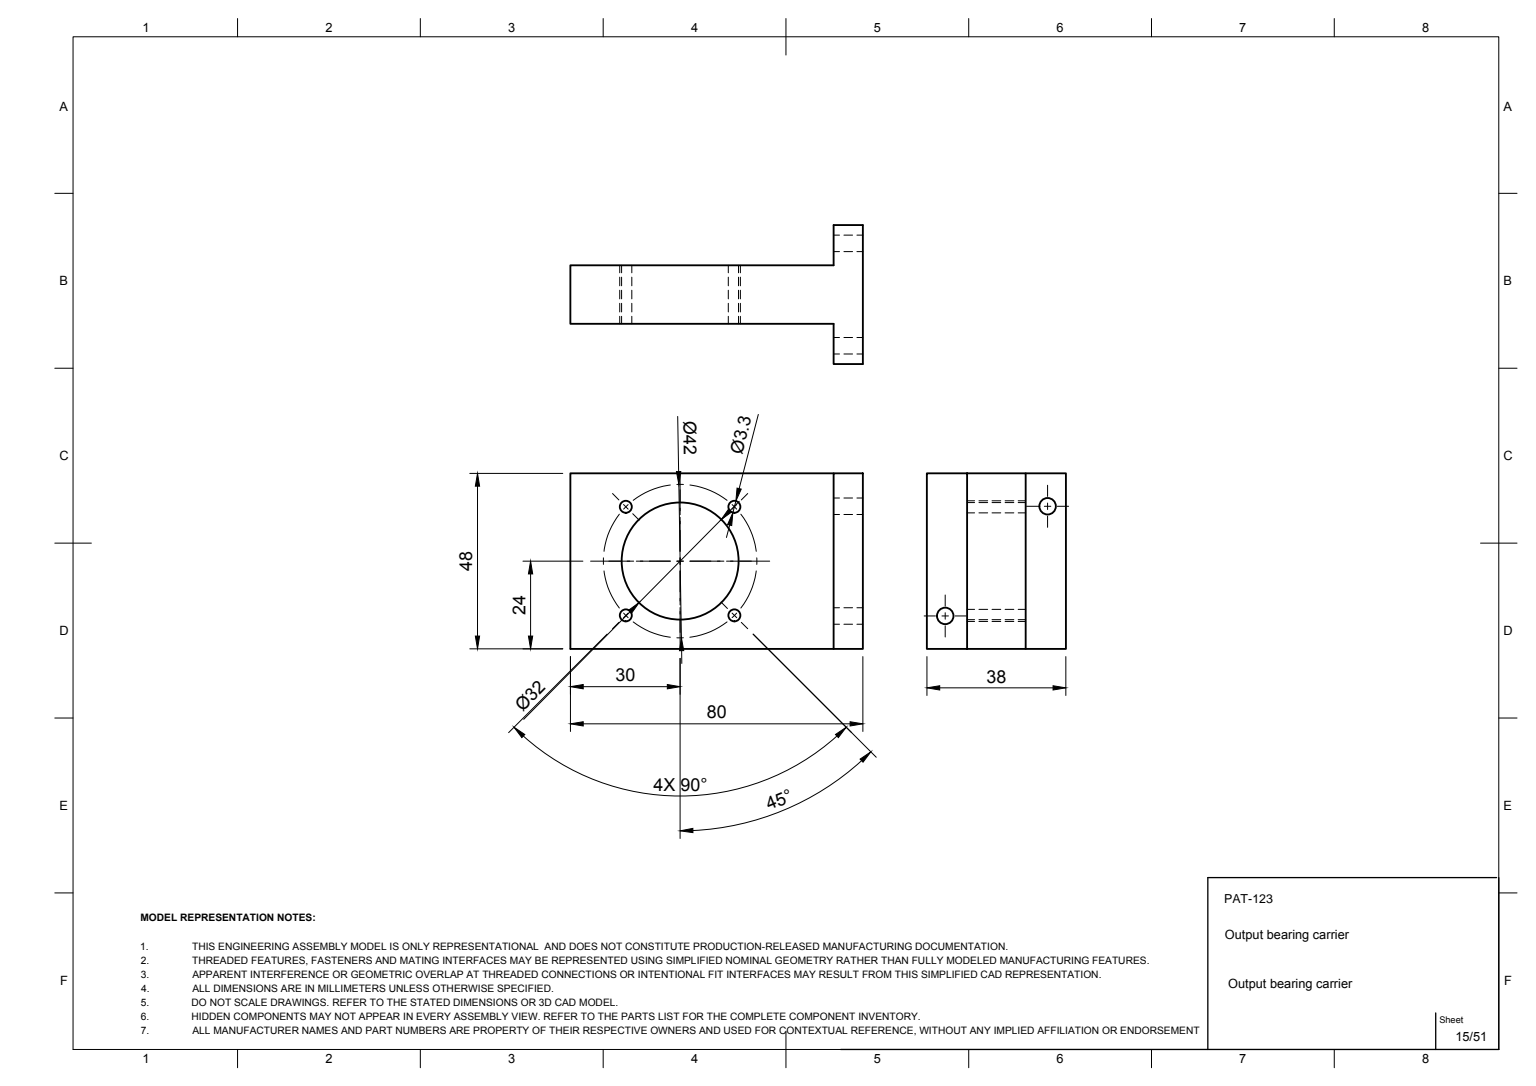
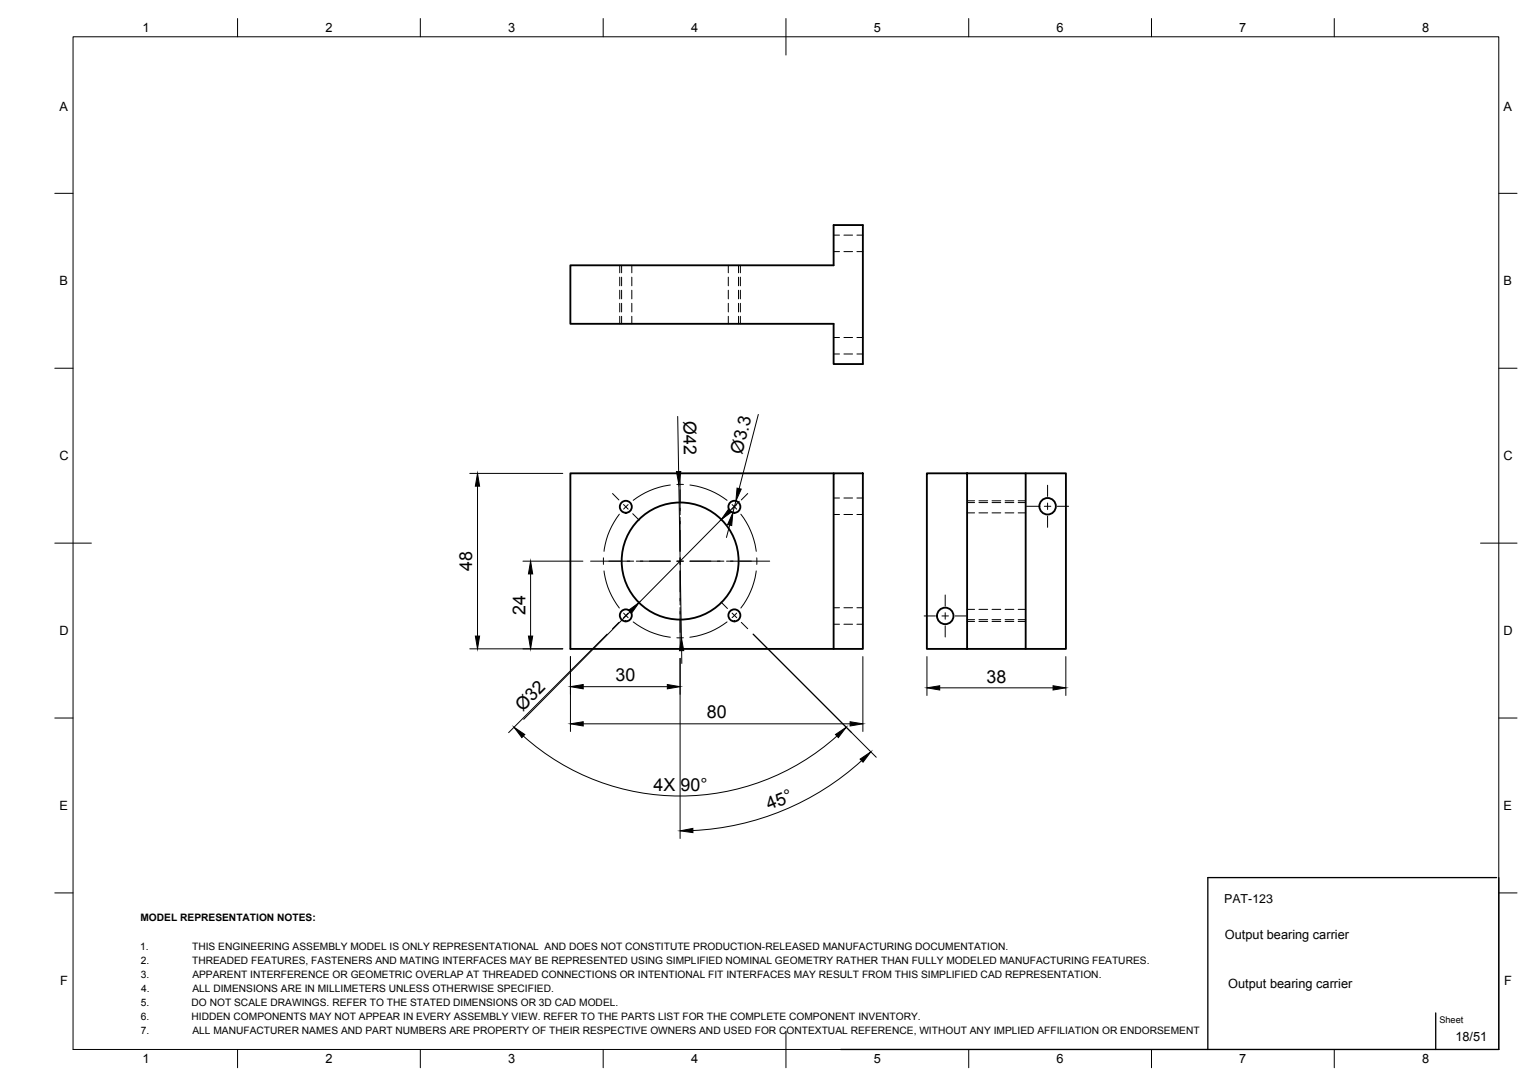
ISO-10303-21;
HEADER;
/* Generated by software containing ST-Developer
 * from STEP Tools, Inc. (www.steptools.com) 
 */

FILE_DESCRIPTION(
/* description */ ('Worm-less right-angle friction wheel drive'),
/* implementation_level */ '2;1');

FILE_NAME(
/* name */ 'Output bearing carrier.step',
/* time_stamp */ '2026-10-28T03:22:36-07:00',
/* author */ (''),
/* organization */ (''),
/* preprocessor_version */ 'ST-DEVELOPER v20.2',
/* originating_system */ 'Autodesk Translation Framework v15.17.0.0',
/* authorisation */ '');

FILE_SCHEMA (('AUTOMOTIVE_DESIGN { 1 0 10303 214 3 1 1 }'));
ENDSEC;

DATA;
#10=MECHANICAL_DESIGN_GEOMETRIC_PRESENTATION_REPRESENTATION('',(#621),#17046);
#527=SHAPE_REPRESENTATION_RELATIONSHIP('SRR','None',#17270,#574);
#574=ADVANCED_BREP_SHAPE_REPRESENTATION('',(#675),#17006);
#621=STYLED_ITEM('',(#17591),#675);
#675=MANIFOLD_SOLID_BREP('Body1',#8176);
#823=FACE_BOUND('',#1918,.T.);
#824=FACE_BOUND('',#1920,.T.);
#825=FACE_BOUND('',#1925,.T.);
#826=FACE_BOUND('',#1926,.T.);
#827=FACE_BOUND('',#1927,.T.);
#828=FACE_BOUND('',#1928,.T.);
#829=FACE_BOUND('',#1929,.T.);
#830=FACE_BOUND('',#1932,.T.);
#831=FACE_BOUND('',#1933,.T.);
#832=FACE_BOUND('',#1934,.T.);
#833=FACE_BOUND('',#1935,.T.);
#834=FACE_BOUND('',#1936,.T.);
#835=FACE_BOUND('',#1939,.T.);
#836=FACE_BOUND('',#1940,.T.);
#1016=PLANE('',#9032);
#1017=PLANE('',#9033);
#1018=PLANE('',#9034);
#1019=PLANE('',#9035);
#1020=PLANE('',#9036);
#1021=PLANE('',#9037);
#1022=PLANE('',#9038);
#1023=PLANE('',#9039);
#1024=PLANE('',#9040);
#1025=PLANE('',#9041);
#1336=FACE_OUTER_BOUND('',#1910,.T.);
#1337=FACE_OUTER_BOUND('',#1911,.T.);
#1338=FACE_OUTER_BOUND('',#1912,.T.);
#1339=FACE_OUTER_BOUND('',#1913,.T.);
#1340=FACE_OUTER_BOUND('',#1914,.T.);
#1341=FACE_OUTER_BOUND('',#1915,.T.);
#1342=FACE_OUTER_BOUND('',#1916,.T.);
#1343=FACE_OUTER_BOUND('',#1917,.T.);
#1344=FACE_OUTER_BOUND('',#1919,.T.);
#1345=FACE_OUTER_BOUND('',#1921,.T.);
#1346=FACE_OUTER_BOUND('',#1922,.T.);
#1347=FACE_OUTER_BOUND('',#1923,.T.);
#1348=FACE_OUTER_BOUND('',#1924,.T.);
#1349=FACE_OUTER_BOUND('',#1930,.T.);
#1350=FACE_OUTER_BOUND('',#1931,.T.);
#1351=FACE_OUTER_BOUND('',#1937,.T.);
#1352=FACE_OUTER_BOUND('',#1938,.T.);
#1910=EDGE_LOOP('',(#6158,#6159,#6160,#6161));
#1911=EDGE_LOOP('',(#6162,#6163,#6164,#6165));
#1912=EDGE_LOOP('',(#6166,#6167,#6168,#6169));
#1913=EDGE_LOOP('',(#6170,#6171,#6172,#6173));
#1914=EDGE_LOOP('',(#6174,#6175,#6176,#6177));
#1915=EDGE_LOOP('',(#6178,#6179,#6180,#6181));
#1916=EDGE_LOOP('',(#6182,#6183,#6184,#6185));
#1917=EDGE_LOOP('',(#6186,#6187,#6188,#6189));
#1918=EDGE_LOOP('',(#6190));
#1919=EDGE_LOOP('',(#6191,#6192,#6193,#6194));
#1920=EDGE_LOOP('',(#6195));
#1921=EDGE_LOOP('',(#6196,#6197,#6198,#6199));
#1922=EDGE_LOOP('',(#6200,#6201,#6202,#6203));
#1923=EDGE_LOOP('',(#6204,#6205,#6206,#6207,#6208,#6209,#6210,#6211));
#1924=EDGE_LOOP('',(#6212,#6213,#6214,#6215));
#1925=EDGE_LOOP('',(#6216));
#1926=EDGE_LOOP('',(#6217));
#1927=EDGE_LOOP('',(#6218));
#1928=EDGE_LOOP('',(#6219));
#1929=EDGE_LOOP('',(#6220));
#1930=EDGE_LOOP('',(#6221,#6222,#6223,#6224,#6225,#6226,#6227,#6228));
#1931=EDGE_LOOP('',(#6229,#6230,#6231,#6232));
#1932=EDGE_LOOP('',(#6233));
#1933=EDGE_LOOP('',(#6234));
#1934=EDGE_LOOP('',(#6235));
#1935=EDGE_LOOP('',(#6236));
#1936=EDGE_LOOP('',(#6237));
#1937=EDGE_LOOP('',(#6238,#6239,#6240,#6241));
#1938=EDGE_LOOP('',(#6242,#6243,#6244,#6245));
#1939=EDGE_LOOP('',(#6246));
#1940=EDGE_LOOP('',(#6247));
#2561=LINE('',#13040,#3101);
#2562=LINE('',#13046,#3102);
#2563=LINE('',#13052,#3103);
#2564=LINE('',#13058,#3104);
#2565=LINE('',#13064,#3105);
#2566=LINE('',#13070,#3106);
#2567=LINE('',#13076,#3107);
#2568=LINE('',#13081,#3108);
#2569=LINE('',#13083,#3109);
#2570=LINE('',#13085,#3110);
#2571=LINE('',#13086,#3111);
#2572=LINE('',#13090,#3112);
#2573=LINE('',#13092,#3113);
#2574=LINE('',#13094,#3114);
#2575=LINE('',#13095,#3115);
#2576=LINE('',#13098,#3116);
#2577=LINE('',#13100,#3117);
#2578=LINE('',#13101,#3118);
#2579=LINE('',#13104,#3119);
#2580=LINE('',#13106,#3120);
#2581=LINE('',#13107,#3121);
#2582=LINE('',#13110,#3122);
#2583=LINE('',#13112,#3123);
#2584=LINE('',#13113,#3124);
#2585=LINE('',#13114,#3125);
#2586=LINE('',#13117,#3126);
#2587=LINE('',#13118,#3127);
#2588=LINE('',#13121,#3128);
#2589=LINE('',#13122,#3129);
#2590=LINE('',#13123,#3130);
#2591=LINE('',#13125,#3131);
#3101=VECTOR('',#10499,0.165);
#3102=VECTOR('',#10506,0.164999999999999);
#3103=VECTOR('',#10513,0.164999999999999);
#3104=VECTOR('',#10520,0.165);
#3105=VECTOR('',#10527,1.6);
#3106=VECTOR('',#10534,0.225);
#3107=VECTOR('',#10541,0.225);
#3108=VECTOR('',#10546,1.);
#3109=VECTOR('',#10547,1.);
#3110=VECTOR('',#10548,1.);
#3111=VECTOR('',#10549,1.);
#3112=VECTOR('',#10552,1.);
#3113=VECTOR('',#10553,1.);
#3114=VECTOR('',#10554,1.);
#3115=VECTOR('',#10555,1.);
#3116=VECTOR('',#10558,1.);
#3117=VECTOR('',#10559,1.);
#3118=VECTOR('',#10560,1.);
#3119=VECTOR('',#10563,1.);
#3120=VECTOR('',#10564,1.);
#3121=VECTOR('',#10565,1.);
#3122=VECTOR('',#10568,1.);
#3123=VECTOR('',#10569,1.);
#3124=VECTOR('',#10570,1.);
#3125=VECTOR('',#10571,1.);
#3126=VECTOR('',#10574,1.);
#3127=VECTOR('',#10575,1.);
#3128=VECTOR('',#10578,1.);
#3129=VECTOR('',#10579,1.);
#3130=VECTOR('',#10580,1.);
#3131=VECTOR('',#10583,1.);
#3585=CIRCLE('',#9012,0.165);
#3586=CIRCLE('',#9013,0.165);
#3587=CIRCLE('',#9015,0.164999999999999);
#3588=CIRCLE('',#9016,0.164999999999999);
#3589=CIRCLE('',#9018,0.164999999999999);
#3590=CIRCLE('',#9019,0.164999999999999);
#3591=CIRCLE('',#9021,0.165);
#3592=CIRCLE('',#9022,0.165);
#3593=CIRCLE('',#9024,1.6);
#3594=CIRCLE('',#9025,1.6);
#3595=CIRCLE('',#9027,0.225);
#3596=CIRCLE('',#9028,0.225);
#3597=CIRCLE('',#9030,0.225);
#3598=CIRCLE('',#9031,0.225);
#4077=VERTEX_POINT('',#13037);
#4078=VERTEX_POINT('',#13039);
#4079=VERTEX_POINT('',#13043);
#4080=VERTEX_POINT('',#13045);
#4081=VERTEX_POINT('',#13049);
#4082=VERTEX_POINT('',#13051);
#4083=VERTEX_POINT('',#13055);
#4084=VERTEX_POINT('',#13057);
#4085=VERTEX_POINT('',#13061);
#4086=VERTEX_POINT('',#13063);
#4087=VERTEX_POINT('',#13067);
#4088=VERTEX_POINT('',#13069);
#4089=VERTEX_POINT('',#13073);
#4090=VERTEX_POINT('',#13075);
#4091=VERTEX_POINT('',#13079);
#4092=VERTEX_POINT('',#13080);
#4093=VERTEX_POINT('',#13082);
#4094=VERTEX_POINT('',#13084);
#4095=VERTEX_POINT('',#13088);
#4096=VERTEX_POINT('',#13089);
#4097=VERTEX_POINT('',#13091);
#4098=VERTEX_POINT('',#13093);
#4099=VERTEX_POINT('',#13097);
#4100=VERTEX_POINT('',#13099);
#4101=VERTEX_POINT('',#13103);
#4102=VERTEX_POINT('',#13105);
#4103=VERTEX_POINT('',#13109);
#4104=VERTEX_POINT('',#13111);
#4105=VERTEX_POINT('',#13116);
#4106=VERTEX_POINT('',#13120);
#4848=EDGE_CURVE('',#4077,#4077,#3585,.T.);
#4849=EDGE_CURVE('',#4077,#4078,#2561,.T.);
#4850=EDGE_CURVE('',#4078,#4078,#3586,.T.);
#4851=EDGE_CURVE('',#4079,#4079,#3587,.T.);
#4852=EDGE_CURVE('',#4079,#4080,#2562,.T.);
#4853=EDGE_CURVE('',#4080,#4080,#3588,.T.);
#4854=EDGE_CURVE('',#4081,#4081,#3589,.T.);
#4855=EDGE_CURVE('',#4081,#4082,#2563,.T.);
#4856=EDGE_CURVE('',#4082,#4082,#3590,.T.);
#4857=EDGE_CURVE('',#4083,#4083,#3591,.T.);
#4858=EDGE_CURVE('',#4083,#4084,#2564,.T.);
#4859=EDGE_CURVE('',#4084,#4084,#3592,.T.);
#4860=EDGE_CURVE('',#4085,#4085,#3593,.T.);
#4861=EDGE_CURVE('',#4085,#4086,#2565,.T.);
#4862=EDGE_CURVE('',#4086,#4086,#3594,.T.);
#4863=EDGE_CURVE('',#4087,#4087,#3595,.T.);
#4864=EDGE_CURVE('',#4087,#4088,#2566,.T.);
#4865=EDGE_CURVE('',#4088,#4088,#3596,.T.);
#4866=EDGE_CURVE('',#4089,#4089,#3597,.T.);
#4867=EDGE_CURVE('',#4089,#4090,#2567,.T.);
#4868=EDGE_CURVE('',#4090,#4090,#3598,.T.);
#4869=EDGE_CURVE('',#4091,#4092,#2568,.T.);
#4870=EDGE_CURVE('',#4093,#4091,#2569,.T.);
#4871=EDGE_CURVE('',#4093,#4094,#2570,.T.);
#4872=EDGE_CURVE('',#4092,#4094,#2571,.T.);
#4873=EDGE_CURVE('',#4095,#4096,#2572,.T.);
#4874=EDGE_CURVE('',#4097,#4095,#2573,.T.);
#4875=EDGE_CURVE('',#4098,#4097,#2574,.T.);
#4876=EDGE_CURVE('',#4096,#4098,#2575,.T.);
#4877=EDGE_CURVE('',#4098,#4099,#2576,.T.);
#4878=EDGE_CURVE('',#4100,#4097,#2577,.T.);
#4879=EDGE_CURVE('',#4099,#4100,#2578,.T.);
#4880=EDGE_CURVE('',#4101,#4093,#2579,.T.);
#4881=EDGE_CURVE('',#4101,#4102,#2580,.T.);
#4882=EDGE_CURVE('',#4094,#4102,#2581,.T.);
#4883=EDGE_CURVE('',#4091,#4103,#2582,.T.);
#4884=EDGE_CURVE('',#4104,#4103,#2583,.T.);
#4885=EDGE_CURVE('',#4096,#4104,#2584,.T.);
#4886=EDGE_CURVE('',#4099,#4101,#2585,.T.);
#4887=EDGE_CURVE('',#4092,#4105,#2586,.T.);
#4888=EDGE_CURVE('',#4103,#4105,#2587,.T.);
#4889=EDGE_CURVE('',#4095,#4106,#2588,.T.);
#4890=EDGE_CURVE('',#4105,#4106,#2589,.T.);
#4891=EDGE_CURVE('',#4102,#4100,#2590,.T.);
#4892=EDGE_CURVE('',#4106,#4104,#2591,.T.);
#6158=ORIENTED_EDGE('',*,*,#4848,.F.);
#6159=ORIENTED_EDGE('',*,*,#4849,.T.);
#6160=ORIENTED_EDGE('',*,*,#4850,.F.);
#6161=ORIENTED_EDGE('',*,*,#4849,.F.);
#6162=ORIENTED_EDGE('',*,*,#4851,.F.);
#6163=ORIENTED_EDGE('',*,*,#4852,.T.);
#6164=ORIENTED_EDGE('',*,*,#4853,.F.);
#6165=ORIENTED_EDGE('',*,*,#4852,.F.);
#6166=ORIENTED_EDGE('',*,*,#4854,.F.);
#6167=ORIENTED_EDGE('',*,*,#4855,.T.);
#6168=ORIENTED_EDGE('',*,*,#4856,.F.);
#6169=ORIENTED_EDGE('',*,*,#4855,.F.);
#6170=ORIENTED_EDGE('',*,*,#4857,.F.);
#6171=ORIENTED_EDGE('',*,*,#4858,.T.);
#6172=ORIENTED_EDGE('',*,*,#4859,.F.);
#6173=ORIENTED_EDGE('',*,*,#4858,.F.);
#6174=ORIENTED_EDGE('',*,*,#4860,.F.);
#6175=ORIENTED_EDGE('',*,*,#4861,.T.);
#6176=ORIENTED_EDGE('',*,*,#4862,.F.);
#6177=ORIENTED_EDGE('',*,*,#4861,.F.);
#6178=ORIENTED_EDGE('',*,*,#4863,.F.);
#6179=ORIENTED_EDGE('',*,*,#4864,.T.);
#6180=ORIENTED_EDGE('',*,*,#4865,.F.);
#6181=ORIENTED_EDGE('',*,*,#4864,.F.);
#6182=ORIENTED_EDGE('',*,*,#4866,.F.);
#6183=ORIENTED_EDGE('',*,*,#4867,.T.);
#6184=ORIENTED_EDGE('',*,*,#4868,.F.);
#6185=ORIENTED_EDGE('',*,*,#4867,.F.);
#6186=ORIENTED_EDGE('',*,*,#4869,.F.);
#6187=ORIENTED_EDGE('',*,*,#4870,.F.);
#6188=ORIENTED_EDGE('',*,*,#4871,.T.);
#6189=ORIENTED_EDGE('',*,*,#4872,.F.);
#6190=ORIENTED_EDGE('',*,*,#4868,.T.);
#6191=ORIENTED_EDGE('',*,*,#4873,.F.);
#6192=ORIENTED_EDGE('',*,*,#4874,.F.);
#6193=ORIENTED_EDGE('',*,*,#4875,.F.);
#6194=ORIENTED_EDGE('',*,*,#4876,.F.);
#6195=ORIENTED_EDGE('',*,*,#4865,.T.);
#6196=ORIENTED_EDGE('',*,*,#4877,.F.);
#6197=ORIENTED_EDGE('',*,*,#4875,.T.);
#6198=ORIENTED_EDGE('',*,*,#4878,.F.);
#6199=ORIENTED_EDGE('',*,*,#4879,.F.);
#6200=ORIENTED_EDGE('',*,*,#4880,.F.);
#6201=ORIENTED_EDGE('',*,*,#4881,.T.);
#6202=ORIENTED_EDGE('',*,*,#4882,.F.);
#6203=ORIENTED_EDGE('',*,*,#4871,.F.);
#6204=ORIENTED_EDGE('',*,*,#4883,.T.);
#6205=ORIENTED_EDGE('',*,*,#4884,.F.);
#6206=ORIENTED_EDGE('',*,*,#4885,.F.);
#6207=ORIENTED_EDGE('',*,*,#4876,.T.);
#6208=ORIENTED_EDGE('',*,*,#4877,.T.);
#6209=ORIENTED_EDGE('',*,*,#4886,.T.);
#6210=ORIENTED_EDGE('',*,*,#4880,.T.);
#6211=ORIENTED_EDGE('',*,*,#4870,.T.);
#6212=ORIENTED_EDGE('',*,*,#4869,.T.);
#6213=ORIENTED_EDGE('',*,*,#4887,.T.);
#6214=ORIENTED_EDGE('',*,*,#4888,.F.);
#6215=ORIENTED_EDGE('',*,*,#4883,.F.);
#6216=ORIENTED_EDGE('',*,*,#4862,.T.);
#6217=ORIENTED_EDGE('',*,*,#4859,.T.);
#6218=ORIENTED_EDGE('',*,*,#4856,.T.);
#6219=ORIENTED_EDGE('',*,*,#4853,.T.);
#6220=ORIENTED_EDGE('',*,*,#4850,.T.);
#6221=ORIENTED_EDGE('',*,*,#4889,.T.);
#6222=ORIENTED_EDGE('',*,*,#4890,.F.);
#6223=ORIENTED_EDGE('',*,*,#4887,.F.);
#6224=ORIENTED_EDGE('',*,*,#4872,.T.);
#6225=ORIENTED_EDGE('',*,*,#4882,.T.);
#6226=ORIENTED_EDGE('',*,*,#4891,.T.);
#6227=ORIENTED_EDGE('',*,*,#4878,.T.);
#6228=ORIENTED_EDGE('',*,*,#4874,.T.);
#6229=ORIENTED_EDGE('',*,*,#4873,.T.);
#6230=ORIENTED_EDGE('',*,*,#4885,.T.);
#6231=ORIENTED_EDGE('',*,*,#4892,.F.);
#6232=ORIENTED_EDGE('',*,*,#4889,.F.);
#6233=ORIENTED_EDGE('',*,*,#4860,.T.);
#6234=ORIENTED_EDGE('',*,*,#4857,.T.);
#6235=ORIENTED_EDGE('',*,*,#4854,.T.);
#6236=ORIENTED_EDGE('',*,*,#4851,.T.);
#6237=ORIENTED_EDGE('',*,*,#4848,.T.);
#6238=ORIENTED_EDGE('',*,*,#4892,.T.);
#6239=ORIENTED_EDGE('',*,*,#4884,.T.);
#6240=ORIENTED_EDGE('',*,*,#4888,.T.);
#6241=ORIENTED_EDGE('',*,*,#4890,.T.);
#6242=ORIENTED_EDGE('',*,*,#4891,.F.);
#6243=ORIENTED_EDGE('',*,*,#4881,.F.);
#6244=ORIENTED_EDGE('',*,*,#4886,.F.);
#6245=ORIENTED_EDGE('',*,*,#4879,.T.);
#6246=ORIENTED_EDGE('',*,*,#4863,.T.);
#6247=ORIENTED_EDGE('',*,*,#4866,.T.);
#7594=CYLINDRICAL_SURFACE('',#9011,0.165);
#7595=CYLINDRICAL_SURFACE('',#9014,0.164999999999999);
#7596=CYLINDRICAL_SURFACE('',#9017,0.164999999999999);
#7597=CYLINDRICAL_SURFACE('',#9020,0.165);
#7598=CYLINDRICAL_SURFACE('',#9023,1.6);
#7599=CYLINDRICAL_SURFACE('',#9026,0.225);
#7600=CYLINDRICAL_SURFACE('',#9029,0.225);
#7828=ADVANCED_FACE('',(#1336),#7594,.F.);
#7829=ADVANCED_FACE('',(#1337),#7595,.F.);
#7830=ADVANCED_FACE('',(#1338),#7596,.F.);
#7831=ADVANCED_FACE('',(#1339),#7597,.F.);
#7832=ADVANCED_FACE('',(#1340),#7598,.F.);
#7833=ADVANCED_FACE('',(#1341),#7599,.F.);
#7834=ADVANCED_FACE('',(#1342),#7600,.F.);
#7835=ADVANCED_FACE('',(#1343,#823),#1016,.T.);
#7836=ADVANCED_FACE('',(#1344,#824),#1017,.T.);
#7837=ADVANCED_FACE('',(#1345),#1018,.T.);
#7838=ADVANCED_FACE('',(#1346),#1019,.T.);
#7839=ADVANCED_FACE('',(#1347),#1020,.T.);
#7840=ADVANCED_FACE('',(#1348,#825,#826,#827,#828,#829),#1021,.T.);
#7841=ADVANCED_FACE('',(#1349),#1022,.T.);
#7842=ADVANCED_FACE('',(#1350,#830,#831,#832,#833,#834),#1023,.T.);
#7843=ADVANCED_FACE('',(#1351),#1024,.T.);
#7844=ADVANCED_FACE('',(#1352,#835,#836),#1025,.F.);
#8176=CLOSED_SHELL('',(#7828,#7829,#7830,#7831,#7832,#7833,#7834,#7835,
#7836,#7837,#7838,#7839,#7840,#7841,#7842,#7843,#7844));
#9010=AXIS2_PLACEMENT_3D('',#13035,#10493,#10494);
#9011=AXIS2_PLACEMENT_3D('',#13036,#10495,#10496);
#9012=AXIS2_PLACEMENT_3D('',#13038,#10497,#10498);
#9013=AXIS2_PLACEMENT_3D('',#13041,#10500,#10501);
#9014=AXIS2_PLACEMENT_3D('',#13042,#10502,#10503);
#9015=AXIS2_PLACEMENT_3D('',#13044,#10504,#10505);
#9016=AXIS2_PLACEMENT_3D('',#13047,#10507,#10508);
#9017=AXIS2_PLACEMENT_3D('',#13048,#10509,#10510);
#9018=AXIS2_PLACEMENT_3D('',#13050,#10511,#10512);
#9019=AXIS2_PLACEMENT_3D('',#13053,#10514,#10515);
#9020=AXIS2_PLACEMENT_3D('',#13054,#10516,#10517);
#9021=AXIS2_PLACEMENT_3D('',#13056,#10518,#10519);
#9022=AXIS2_PLACEMENT_3D('',#13059,#10521,#10522);
#9023=AXIS2_PLACEMENT_3D('',#13060,#10523,#10524);
#9024=AXIS2_PLACEMENT_3D('',#13062,#10525,#10526);
#9025=AXIS2_PLACEMENT_3D('',#13065,#10528,#10529);
#9026=AXIS2_PLACEMENT_3D('',#13066,#10530,#10531);
#9027=AXIS2_PLACEMENT_3D('',#13068,#10532,#10533);
#9028=AXIS2_PLACEMENT_3D('',#13071,#10535,#10536);
#9029=AXIS2_PLACEMENT_3D('',#13072,#10537,#10538);
#9030=AXIS2_PLACEMENT_3D('',#13074,#10539,#10540);
#9031=AXIS2_PLACEMENT_3D('',#13077,#10542,#10543);
#9032=AXIS2_PLACEMENT_3D('',#13078,#10544,#10545);
#9033=AXIS2_PLACEMENT_3D('',#13087,#10550,#10551);
#9034=AXIS2_PLACEMENT_3D('',#13096,#10556,#10557);
#9035=AXIS2_PLACEMENT_3D('',#13102,#10561,#10562);
#9036=AXIS2_PLACEMENT_3D('',#13108,#10566,#10567);
#9037=AXIS2_PLACEMENT_3D('',#13115,#10572,#10573);
#9038=AXIS2_PLACEMENT_3D('',#13119,#10576,#10577);
#9039=AXIS2_PLACEMENT_3D('',#13124,#10581,#10582);
#9040=AXIS2_PLACEMENT_3D('',#13126,#10584,#10585);
#9041=AXIS2_PLACEMENT_3D('',#13127,#10586,#10587);
#10493=DIRECTION('axis',(0.,0.,1.));
#10494=DIRECTION('refdir',(1.,0.,0.));
#10495=DIRECTION('center_axis',(1.,0.,0.));
#10496=DIRECTION('ref_axis',(0.,0.,-1.));
#10497=DIRECTION('center_axis',(1.,0.,0.));
#10498=DIRECTION('ref_axis',(0.,0.,-1.));
#10499=DIRECTION('',(1.,0.,0.));
#10500=DIRECTION('center_axis',(-1.,0.,0.));
#10501=DIRECTION('ref_axis',(0.,0.,-1.));
#10502=DIRECTION('center_axis',(1.,0.,0.));
#10503=DIRECTION('ref_axis',(0.,0.,-1.));
#10504=DIRECTION('center_axis',(1.,0.,0.));
#10505=DIRECTION('ref_axis',(0.,0.,-1.));
#10506=DIRECTION('',(1.,0.,0.));
#10507=DIRECTION('center_axis',(-1.,0.,0.));
#10508=DIRECTION('ref_axis',(0.,0.,-1.));
#10509=DIRECTION('center_axis',(1.,0.,0.));
#10510=DIRECTION('ref_axis',(0.,0.,-1.));
#10511=DIRECTION('center_axis',(1.,0.,0.));
#10512=DIRECTION('ref_axis',(0.,0.,-1.));
#10513=DIRECTION('',(1.,0.,0.));
#10514=DIRECTION('center_axis',(-1.,0.,0.));
#10515=DIRECTION('ref_axis',(0.,0.,-1.));
#10516=DIRECTION('center_axis',(1.,0.,0.));
#10517=DIRECTION('ref_axis',(0.,0.,-1.));
#10518=DIRECTION('center_axis',(1.,0.,0.));
#10519=DIRECTION('ref_axis',(0.,0.,-1.));
#10520=DIRECTION('',(1.,0.,0.));
#10521=DIRECTION('center_axis',(-1.,0.,0.));
#10522=DIRECTION('ref_axis',(0.,0.,-1.));
#10523=DIRECTION('center_axis',(1.,0.,0.));
#10524=DIRECTION('ref_axis',(0.,0.,-1.));
#10525=DIRECTION('center_axis',(1.,0.,0.));
#10526=DIRECTION('ref_axis',(0.,0.,-1.));
#10527=DIRECTION('',(1.,0.,0.));
#10528=DIRECTION('center_axis',(-1.,0.,0.));
#10529=DIRECTION('ref_axis',(0.,0.,-1.));
#10530=DIRECTION('center_axis',(0.,0.,1.));
#10531=DIRECTION('ref_axis',(1.,0.,0.));
#10532=DIRECTION('center_axis',(0.,0.,1.));
#10533=DIRECTION('ref_axis',(1.,0.,0.));
#10534=DIRECTION('',(0.,0.,1.));
#10535=DIRECTION('center_axis',(0.,0.,-1.));
#10536=DIRECTION('ref_axis',(1.,0.,0.));
#10537=DIRECTION('center_axis',(0.,0.,1.));
#10538=DIRECTION('ref_axis',(1.,0.,0.));
#10539=DIRECTION('center_axis',(0.,0.,1.));
#10540=DIRECTION('ref_axis',(1.,0.,0.));
#10541=DIRECTION('',(0.,0.,1.));
#10542=DIRECTION('center_axis',(0.,0.,-1.));
#10543=DIRECTION('ref_axis',(1.,0.,0.));
#10544=DIRECTION('center_axis',(0.,0.,1.));
#10545=DIRECTION('ref_axis',(1.,0.,0.));
#10546=DIRECTION('',(0.,1.,0.));
#10547=DIRECTION('',(-1.,0.,0.));
#10548=DIRECTION('',(0.,1.,0.));
#10549=DIRECTION('',(1.,0.,0.));
#10550=DIRECTION('center_axis',(0.,0.,1.));
#10551=DIRECTION('ref_axis',(1.,0.,0.));
#10552=DIRECTION('',(0.,-1.,0.));
#10553=DIRECTION('',(1.,0.,0.));
#10554=DIRECTION('',(0.,1.,0.));
#10555=DIRECTION('',(-1.,0.,0.));
#10556=DIRECTION('center_axis',(-1.,0.,0.));
#10557=DIRECTION('ref_axis',(0.,0.,1.));
#10558=DIRECTION('',(0.,0.,-1.));
#10559=DIRECTION('',(0.,0.,1.));
#10560=DIRECTION('',(0.,1.,0.));
#10561=DIRECTION('center_axis',(1.,0.,0.));
#10562=DIRECTION('ref_axis',(0.,0.,-1.));
#10563=DIRECTION('',(0.,0.,1.));
#10564=DIRECTION('',(0.,1.,0.));
#10565=DIRECTION('',(0.,0.,-1.));
#10566=DIRECTION('center_axis',(0.,-1.,0.));
#10567=DIRECTION('ref_axis',(1.,0.,0.));
#10568=DIRECTION('',(0.,0.,1.));
#10569=DIRECTION('',(1.,0.,0.));
#10570=DIRECTION('',(0.,0.,1.));
#10571=DIRECTION('',(1.,0.,0.));
#10572=DIRECTION('center_axis',(1.,0.,0.));
#10573=DIRECTION('ref_axis',(0.,1.,0.));
#10574=DIRECTION('',(0.,0.,1.));
#10575=DIRECTION('',(0.,1.,0.));
#10576=DIRECTION('center_axis',(0.,1.,0.));
#10577=DIRECTION('ref_axis',(-1.,0.,0.));
#10578=DIRECTION('',(0.,0.,1.));
#10579=DIRECTION('',(-1.,0.,0.));
#10580=DIRECTION('',(-1.,0.,0.));
#10581=DIRECTION('center_axis',(-1.,0.,0.));
#10582=DIRECTION('ref_axis',(0.,-1.,0.));
#10583=DIRECTION('',(0.,-1.,0.));
#10584=DIRECTION('center_axis',(0.,0.,1.));
#10585=DIRECTION('ref_axis',(1.,0.,0.));
#10586=DIRECTION('center_axis',(0.,0.,1.));
#10587=DIRECTION('ref_axis',(1.,0.,0.));
#13035=CARTESIAN_POINT('',(0.,0.,0.));
#13036=CARTESIAN_POINT('Origin',(-1.2,1.51507575950825,5.51507575950825));
#13037=CARTESIAN_POINT('',(-1.1,1.51507575950825,5.68007575950825));
#13038=CARTESIAN_POINT('Origin',(-1.1,1.51507575950825,5.51507575950825));
#13039=CARTESIAN_POINT('',(0.5,1.51507575950825,5.68007575950825));
#13040=CARTESIAN_POINT('',(-1.2,1.51507575950825,5.68007575950825));
#13041=CARTESIAN_POINT('Origin',(0.5,1.51507575950825,5.51507575950825));
#13042=CARTESIAN_POINT('Origin',(-1.2,1.51507575950825,8.48492424049175));
#13043=CARTESIAN_POINT('',(-1.1,1.51507575950825,8.64992424049175));
#13044=CARTESIAN_POINT('Origin',(-1.1,1.51507575950825,8.48492424049175));
#13045=CARTESIAN_POINT('',(0.5,1.51507575950825,8.64992424049175));
#13046=CARTESIAN_POINT('',(-1.2,1.51507575950825,8.64992424049175));
#13047=CARTESIAN_POINT('Origin',(0.5,1.51507575950825,8.48492424049175));
#13048=CARTESIAN_POINT('Origin',(-1.2,4.48492424049175,8.48492424049175));
#13049=CARTESIAN_POINT('',(-1.1,4.48492424049175,8.64992424049175));
#13050=CARTESIAN_POINT('Origin',(-1.1,4.48492424049175,8.48492424049175));
#13051=CARTESIAN_POINT('',(0.5,4.48492424049175,8.64992424049175));
#13052=CARTESIAN_POINT('',(-1.2,4.48492424049175,8.64992424049175));
#13053=CARTESIAN_POINT('Origin',(0.5,4.48492424049175,8.48492424049175));
#13054=CARTESIAN_POINT('Origin',(-1.2,4.48492424049175,5.51507575950825));
#13055=CARTESIAN_POINT('',(-1.1,4.48492424049175,5.68007575950825));
#13056=CARTESIAN_POINT('Origin',(-1.1,4.48492424049175,5.51507575950825));
#13057=CARTESIAN_POINT('',(0.5,4.48492424049175,5.68007575950825));
#13058=CARTESIAN_POINT('',(-1.2,4.48492424049175,5.68007575950825));
#13059=CARTESIAN_POINT('Origin',(0.5,4.48492424049175,5.51507575950825));
#13060=CARTESIAN_POINT('Origin',(-1.2,3.,7.));
#13061=CARTESIAN_POINT('',(-1.1,3.,8.6));
#13062=CARTESIAN_POINT('Origin',(-1.1,3.,7.));
#13063=CARTESIAN_POINT('',(0.5,3.,8.6));
#13064=CARTESIAN_POINT('',(-1.2,3.,8.6));
#13065=CARTESIAN_POINT('Origin',(0.5,3.,7.));
#13066=CARTESIAN_POINT('Origin',(-1.7,1.5,1.9));
#13067=CARTESIAN_POINT('',(-1.925,1.5,2.));
#13068=CARTESIAN_POINT('Origin',(-1.7,1.5,2.));
#13069=CARTESIAN_POINT('',(-1.925,1.5,2.8));
#13070=CARTESIAN_POINT('',(-1.925,1.5,1.9));
#13071=CARTESIAN_POINT('Origin',(-1.7,1.5,2.8));
#13072=CARTESIAN_POINT('Origin',(1.1,4.5,1.9));
#13073=CARTESIAN_POINT('',(0.875,4.5,2.));
#13074=CARTESIAN_POINT('Origin',(1.1,4.5,2.));
#13075=CARTESIAN_POINT('',(0.875,4.5,2.8));
#13076=CARTESIAN_POINT('',(0.875,4.5,1.9));
#13077=CARTESIAN_POINT('Origin',(1.1,4.5,2.8));
#13078=CARTESIAN_POINT('Origin',(-2.2,0.6,2.8));
#13079=CARTESIAN_POINT('',(0.5,0.6,2.8));
#13080=CARTESIAN_POINT('',(0.5,5.4,2.8));
#13081=CARTESIAN_POINT('',(0.5,0.6,2.8));
#13082=CARTESIAN_POINT('',(1.6,0.6,2.8));
#13083=CARTESIAN_POINT('',(1.6,0.6,2.8));
#13084=CARTESIAN_POINT('',(1.6,5.4,2.8));
#13085=CARTESIAN_POINT('',(1.6,0.6,2.8));
#13086=CARTESIAN_POINT('',(1.6,5.4,2.8));
#13087=CARTESIAN_POINT('Origin',(-2.2,0.6,2.8));
#13088=CARTESIAN_POINT('',(-1.1,5.4,2.8));
#13089=CARTESIAN_POINT('',(-1.1,0.6,2.8));
#13090=CARTESIAN_POINT('',(-1.1,3.,2.8));
#13091=CARTESIAN_POINT('',(-2.2,5.4,2.8));
#13092=CARTESIAN_POINT('',(1.6,5.4,2.8));
#13093=CARTESIAN_POINT('',(-2.2,0.6,2.8));
#13094=CARTESIAN_POINT('',(-2.2,0.6,2.8));
#13095=CARTESIAN_POINT('',(1.6,0.6,2.8));
#13096=CARTESIAN_POINT('Origin',(-2.2,0.6,2.));
#13097=CARTESIAN_POINT('',(-2.2,0.6,2.));
#13098=CARTESIAN_POINT('',(-2.2,0.6,2.8));
#13099=CARTESIAN_POINT('',(-2.2,5.4,2.));
#13100=CARTESIAN_POINT('',(-2.2,5.4,2.8));
#13101=CARTESIAN_POINT('',(-2.2,0.6,2.));
#13102=CARTESIAN_POINT('Origin',(1.6,0.6,2.8));
#13103=CARTESIAN_POINT('',(1.6,0.6,2.));
#13104=CARTESIAN_POINT('',(1.6,0.6,2.));
#13105=CARTESIAN_POINT('',(1.6,5.4,2.));
#13106=CARTESIAN_POINT('',(1.6,0.6,2.));
#13107=CARTESIAN_POINT('',(1.6,5.4,2.));
#13108=CARTESIAN_POINT('Origin',(-1.1,0.6,2.));
#13109=CARTESIAN_POINT('',(0.5,0.6,10.));
#13110=CARTESIAN_POINT('',(0.5,0.6,2.));
#13111=CARTESIAN_POINT('',(-1.1,0.6,10.));
#13112=CARTESIAN_POINT('',(-1.1,0.6,10.));
#13113=CARTESIAN_POINT('',(-1.1,0.6,2.));
#13114=CARTESIAN_POINT('',(-2.2,0.6,2.));
#13115=CARTESIAN_POINT('Origin',(0.5,0.6,2.));
#13116=CARTESIAN_POINT('',(0.5,5.4,10.));
#13117=CARTESIAN_POINT('',(0.5,5.4,2.));
#13118=CARTESIAN_POINT('',(0.5,0.6,10.));
#13119=CARTESIAN_POINT('Origin',(0.5,5.4,2.));
#13120=CARTESIAN_POINT('',(-1.1,5.4,10.));
#13121=CARTESIAN_POINT('',(-1.1,5.4,2.));
#13122=CARTESIAN_POINT('',(0.5,5.4,10.));
#13123=CARTESIAN_POINT('',(-2.2,5.4,2.));
#13124=CARTESIAN_POINT('Origin',(-1.1,5.4,2.));
#13125=CARTESIAN_POINT('',(-1.1,5.4,10.));
#13126=CARTESIAN_POINT('Origin',(-0.3,3.,10.));
#13127=CARTESIAN_POINT('Origin',(-0.3,3.,2.));
#16953=UNCERTAINTY_MEASURE_WITH_UNIT(LENGTH_MEASURE(0.001),#17047,
'DISTANCE_ACCURACY_VALUE',
'Maximum model space distance between geometric entities at asserted c
onnectivities');
#16993=UNCERTAINTY_MEASURE_WITH_UNIT(LENGTH_MEASURE(0.001),#17047,
'DISTANCE_ACCURACY_VALUE',
'Maximum model space distance between geometric entities at asserted c
onnectivities');
#17006=(
GEOMETRIC_REPRESENTATION_CONTEXT(3)
GLOBAL_UNCERTAINTY_ASSIGNED_CONTEXT((#16953))
GLOBAL_UNIT_ASSIGNED_CONTEXT((#17047,#17049,#17050))
REPRESENTATION_CONTEXT('','3D')
);
#17046=(
GEOMETRIC_REPRESENTATION_CONTEXT(3)
GLOBAL_UNCERTAINTY_ASSIGNED_CONTEXT((#16993))
GLOBAL_UNIT_ASSIGNED_CONTEXT((#17047,#17049,#17050))
REPRESENTATION_CONTEXT('','3D')
);
#17047=(
LENGTH_UNIT()
NAMED_UNIT(*)
SI_UNIT(.CENTI.,.METRE.)
);
#17049=(
NAMED_UNIT(*)
PLANE_ANGLE_UNIT()
SI_UNIT($,.RADIAN.)
);
#17050=(
NAMED_UNIT(*)
SI_UNIT($,.STERADIAN.)
SOLID_ANGLE_UNIT()
);
#17063=SHAPE_DEFINITION_REPRESENTATION(#17115,#17270);
#17115=PRODUCT_DEFINITION_SHAPE('',$,#17323);
#17270=SHAPE_REPRESENTATION('',(#9010),#17006);
#17310=PRODUCT_DEFINITION_CONTEXT('part definition',#17468,'design');
#17323=PRODUCT_DEFINITION('Output bearing carrier',
'Output bearing carrier',#17375,#17310);
#17375=PRODUCT_DEFINITION_FORMATION('',$,#17482);
#17468=APPLICATION_CONTEXT(
'Core Data for Automotive Mechanical Design Process');
#17469=PRODUCT_CONTEXT('part definition',#17468,'mechanical');
#17482=PRODUCT('Output bearing carrier','Output bearing carrier',
'Output bearing carrier',(#17469));
#17585=COLOUR_RGB('Grey',0.48,0.52,0.57);
#17586=FILL_AREA_STYLE_COLOUR('',#17585);
#17587=FILL_AREA_STYLE('',(#17586));
#17588=SURFACE_STYLE_FILL_AREA(#17587);
#17589=SURFACE_SIDE_STYLE('',(#17588));
#17590=SURFACE_STYLE_USAGE(.BOTH.,#17589);
#17591=PRESENTATION_STYLE_ASSIGNMENT((#17590));
ENDSEC;
END-ISO-10303-21;
